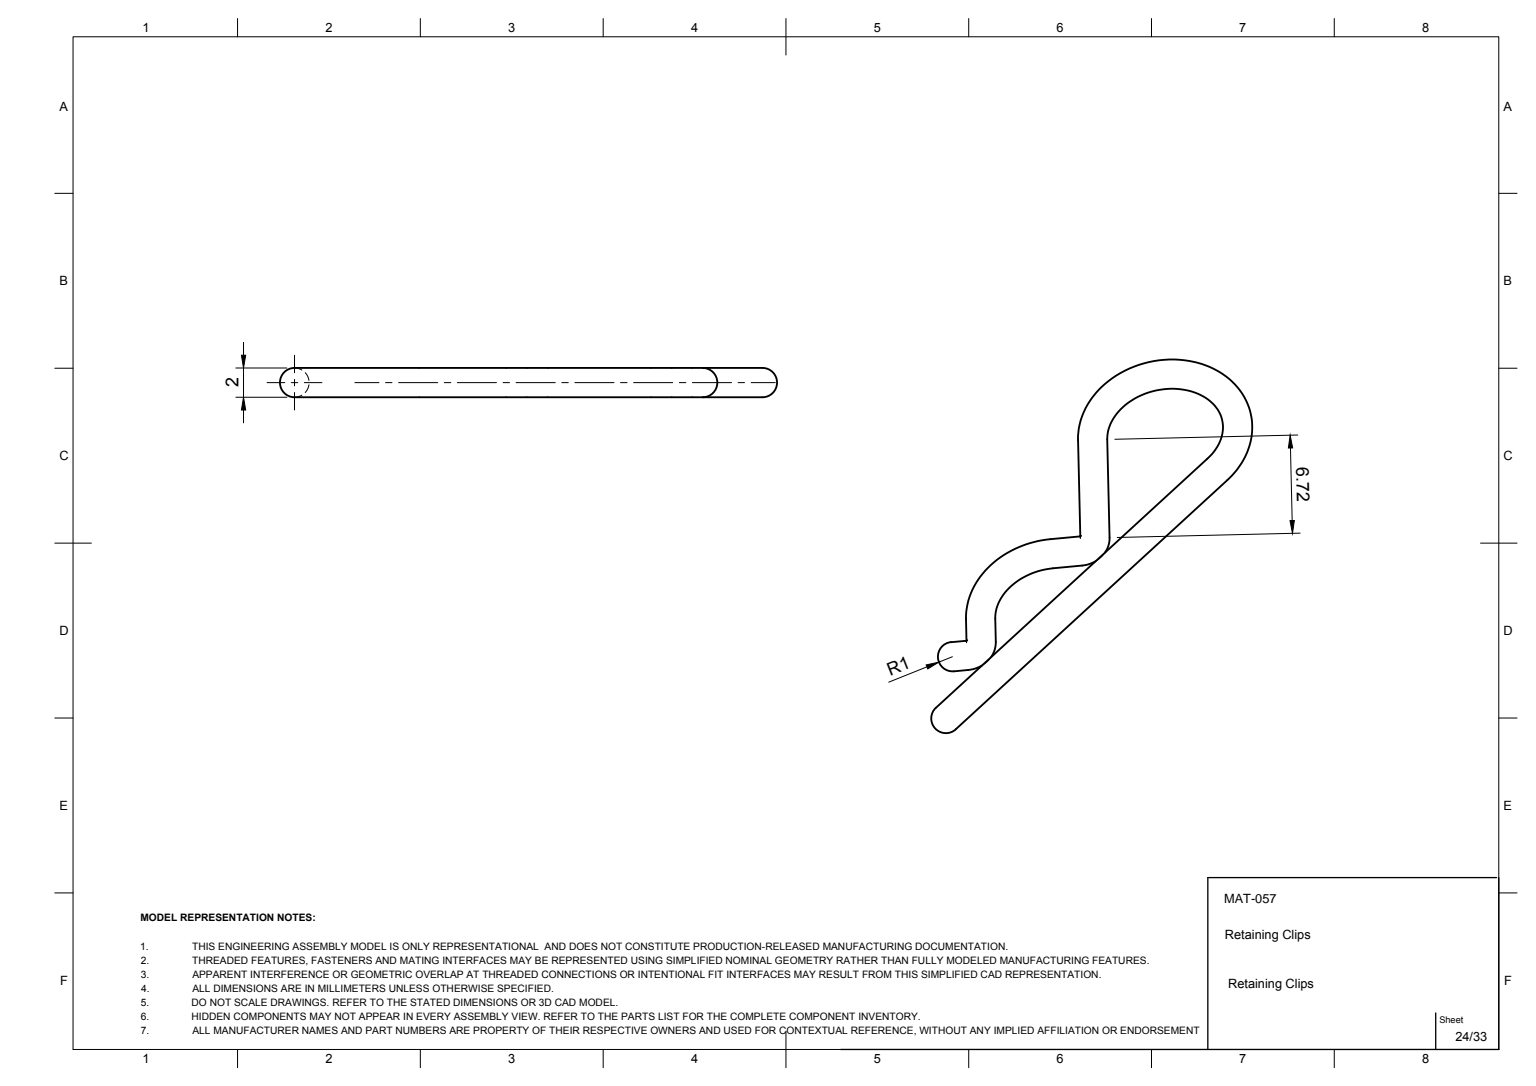
ISO-10303-21;
HEADER;
/* Generated by software containing ST-Developer
 * from STEP Tools, Inc. (www.steptools.com) 
 */

FILE_DESCRIPTION(
/* description */ ('STEP AP214', 'CAx-IF Rec.Pracs.---Representation and Presentation of Product Manufa
cturing Information (PMI)---4.0---2014-10-13'),
/* implementation_level */ '2;1');

FILE_NAME(
/* name */ 'Retaining Clips.step',
/* time_stamp */ '2026-10-28T23:34:22+01:00',
/* author */ (''),
/* organization */ (''),
/* preprocessor_version */ 'ST-DEVELOPER v20.2',
/* originating_system */ 'Autodesk Translation Framework v15.17.0.0',
/* authorisation */ '');

FILE_SCHEMA (('AP242_MANAGED_MODEL_BASED_3D_ENGINEERING_MIM_LF { 1 0 10303 442 2 1 4 }'));
ENDSEC;

DATA;
#10=MECHANICAL_DESIGN_GEOMETRIC_PRESENTATION_REPRESENTATION('',(#266,#267),#27807);
#219=SHAPE_REPRESENTATION_RELATIONSHIP('SRR','None',#27916,#241);
#241=ADVANCED_BREP_SHAPE_REPRESENTATION('',(#295,#296),#27796);
#266=STYLED_ITEM('',(#28070),#295);
#267=STYLED_ITEM('',(#28070),#296);
#295=MANIFOLD_SOLID_BREP('Body1',#12042);
#296=MANIFOLD_SOLID_BREP('Body2',#12043);
#318=(
BOUNDED_SURFACE()
B_SPLINE_SURFACE(2,2,((#22381,#22382,#22383),(#22384,#22385,#22386),(#22387,
#22388,#22389),(#22390,#22391,#22392),(#22393,#22394,#22395),(#22396,#22397,
#22398),(#22399,#22400,#22401),(#22402,#22403,#22404),(#22405,#22406,#22407)),
 .UNSPECIFIED.,.T.,.F.,.F.)
B_SPLINE_SURFACE_WITH_KNOTS((3,2,2,2,3),(3,3),(-3.14159265358979,-1.5707963267949,
0.,1.5707963267949,3.14159265358979),(-2.35619449019236,-0.785398163397175),
 .UNSPECIFIED.)
GEOMETRIC_REPRESENTATION_ITEM()
RATIONAL_B_SPLINE_SURFACE(((1.,0.707106781186444,1.),(0.707106781186499,
0.499999999999893,0.707106781186499),(1.,0.707106781186444,1.),(0.707106781186553,
0.499999999999931,0.707106781186553),(1.,0.707106781186444,1.),(0.707106781186499,
0.499999999999893,0.707106781186499),(1.,0.707106781186444,1.),(0.707106781186553,
0.499999999999931,0.707106781186553),(1.,0.707106781186444,1.)))
REPRESENTATION_ITEM('')
SURFACE()
);
#319=(
BOUNDED_SURFACE()
B_SPLINE_SURFACE(2,2,((#22408,#22409,#22410),(#22411,#22412,#22413),(#22414,
#22415,#22416),(#22417,#22418,#22419),(#22420,#22421,#22422),(#22423,#22424,
#22425),(#22426,#22427,#22428),(#22429,#22430,#22431),(#22432,#22433,#22434)),
 .UNSPECIFIED.,.T.,.F.,.F.)
B_SPLINE_SURFACE_WITH_KNOTS((3,2,2,2,3),(3,3),(-3.14159265358979,-1.5707963267949,
0.,1.5707963267949,3.14159265358979),(-2.35619449019277,-0.785398163397194),
 .UNSPECIFIED.)
GEOMETRIC_REPRESENTATION_ITEM()
RATIONAL_B_SPLINE_SURFACE(((1.,0.707106781186307,1.),(0.707106781186516,
0.499999999999808,0.707106781186516),(1.,0.707106781186307,1.),(0.707106781186497,
0.499999999999794,0.707106781186497),(1.,0.707106781186307,1.),(0.707106781186516,
0.499999999999808,0.707106781186516),(1.,0.707106781186307,1.),(0.707106781186497,
0.499999999999794,0.707106781186497),(1.,0.707106781186307,1.)))
REPRESENTATION_ITEM('')
SURFACE()
);
#320=(
BOUNDED_SURFACE()
B_SPLINE_SURFACE(2,2,((#22485,#22486,#22487),(#22488,#22489,#22490),(#22491,
#22492,#22493),(#22494,#22495,#22496),(#22497,#22498,#22499),(#22500,#22501,
#22502),(#22503,#22504,#22505),(#22506,#22507,#22508),(#22509,#22510,#22511)),
 .UNSPECIFIED.,.T.,.F.,.F.)
B_SPLINE_SURFACE_WITH_KNOTS((3,2,2,2,3),(3,3),(-3.14159265358979,-1.5707963267949,
0.,1.5707963267949,3.14159265358979),(-2.35619449019236,-0.785398163397439),
 .UNSPECIFIED.)
GEOMETRIC_REPRESENTATION_ITEM()
RATIONAL_B_SPLINE_SURFACE(((1.,0.707106781186539,1.),(0.707106781186531,
0.499999999999982,0.707106781186531),(1.,0.707106781186539,1.),(0.707106781186538,
0.499999999999987,0.707106781186538),(1.,0.707106781186539,1.),(0.707106781186531,
0.499999999999982,0.707106781186531),(1.,0.707106781186539,1.),(0.707106781186538,
0.499999999999987,0.707106781186538),(1.,0.707106781186539,1.)))
REPRESENTATION_ITEM('')
SURFACE()
);
#321=(
BOUNDED_SURFACE()
B_SPLINE_SURFACE(2,2,((#22512,#22513,#22514),(#22515,#22516,#22517),(#22518,
#22519,#22520),(#22521,#22522,#22523),(#22524,#22525,#22526),(#22527,#22528,
#22529),(#22530,#22531,#22532),(#22533,#22534,#22535),(#22536,#22537,#22538)),
 .UNSPECIFIED.,.T.,.F.,.F.)
B_SPLINE_SURFACE_WITH_KNOTS((3,2,2,2,3),(3,3),(-3.14159265358979,-1.5707963267949,
0.,1.5707963267949,3.14159265358979),(-2.35619449019241,-0.785398163397432),
 .UNSPECIFIED.)
GEOMETRIC_REPRESENTATION_ITEM()
RATIONAL_B_SPLINE_SURFACE(((1.,0.707106781186519,1.),(0.707106781186627,
0.500000000000036,0.707106781186627),(1.,0.707106781186519,1.),(0.707106781186571,
0.499999999999996,0.707106781186571),(1.,0.707106781186519,1.),(0.707106781186627,
0.500000000000036,0.707106781186627),(1.,0.707106781186519,1.),(0.707106781186571,
0.499999999999996,0.707106781186571),(1.,0.707106781186519,1.)))
REPRESENTATION_ITEM('')
SURFACE()
);
#331=SPHERICAL_SURFACE('',#13311,1.);
#332=SPHERICAL_SURFACE('',#13315,1.);
#333=SPHERICAL_SURFACE('',#13340,1.);
#334=SPHERICAL_SURFACE('',#13344,1.);
#834=TOROIDAL_SURFACE('',#13303,5.00000000000001,1.);
#835=TOROIDAL_SURFACE('',#13307,5.,1.);
#836=TOROIDAL_SURFACE('',#13332,5.00000000000001,1.);
#837=TOROIDAL_SURFACE('',#13336,5.,1.);
#1157=CYLINDRICAL_SURFACE('',#13319,0.999999999999997);
#1158=CYLINDRICAL_SURFACE('',#13322,0.999999999999983);
#1159=CYLINDRICAL_SURFACE('',#13325,0.999999999999997);
#1160=CYLINDRICAL_SURFACE('',#13328,1.00000000000002);
#1161=CYLINDRICAL_SURFACE('',#13331,1.00000000000002);
#1162=CYLINDRICAL_SURFACE('',#13348,1.);
#1163=CYLINDRICAL_SURFACE('',#13351,0.999999999999989);
#1164=CYLINDRICAL_SURFACE('',#13354,1.);
#1165=CYLINDRICAL_SURFACE('',#13357,0.999999999999999);
#1166=CYLINDRICAL_SURFACE('',#13360,0.999999999999993);
#1732=FACE_OUTER_BOUND('',#2510,.T.);
#1733=FACE_OUTER_BOUND('',#2511,.T.);
#1734=FACE_OUTER_BOUND('',#2512,.T.);
#1735=FACE_OUTER_BOUND('',#2513,.T.);
#1736=FACE_OUTER_BOUND('',#2514,.T.);
#1737=FACE_OUTER_BOUND('',#2515,.T.);
#1738=FACE_OUTER_BOUND('',#2516,.T.);
#1739=FACE_OUTER_BOUND('',#2517,.T.);
#1740=FACE_OUTER_BOUND('',#2518,.T.);
#1741=FACE_OUTER_BOUND('',#2519,.T.);
#1742=FACE_OUTER_BOUND('',#2520,.T.);
#1743=FACE_OUTER_BOUND('',#2521,.T.);
#1744=FACE_OUTER_BOUND('',#2522,.T.);
#1745=FACE_OUTER_BOUND('',#2523,.T.);
#1746=FACE_OUTER_BOUND('',#2524,.T.);
#1747=FACE_OUTER_BOUND('',#2525,.T.);
#1748=FACE_OUTER_BOUND('',#2526,.T.);
#1749=FACE_OUTER_BOUND('',#2527,.T.);
#1750=FACE_OUTER_BOUND('',#2528,.T.);
#1751=FACE_OUTER_BOUND('',#2529,.T.);
#1752=FACE_OUTER_BOUND('',#2530,.T.);
#1753=FACE_OUTER_BOUND('',#2531,.T.);
#2510=EDGE_LOOP('',(#10271,#10272,#10273,#10274));
#2511=EDGE_LOOP('',(#10275,#10276,#10277,#10278));
#2512=EDGE_LOOP('',(#10279,#10280,#10281,#10282));
#2513=EDGE_LOOP('',(#10283,#10284,#10285,#10286));
#2514=EDGE_LOOP('',(#10287,#10288,#10289,#10290,#10291,#10292));
#2515=EDGE_LOOP('',(#10293,#10294,#10295,#10296,#10297));
#2516=EDGE_LOOP('',(#10298,#10299,#10300,#10301,#10302));
#2517=EDGE_LOOP('',(#10303,#10304,#10305,#10306,#10307));
#2518=EDGE_LOOP('',(#10308,#10309,#10310,#10311,#10312));
#2519=EDGE_LOOP('',(#10313,#10314,#10315,#10316));
#2520=EDGE_LOOP('',(#10317,#10318,#10319,#10320));
#2521=EDGE_LOOP('',(#10321,#10322,#10323,#10324));
#2522=EDGE_LOOP('',(#10325,#10326,#10327,#10328));
#2523=EDGE_LOOP('',(#10329,#10330,#10331,#10332));
#2524=EDGE_LOOP('',(#10333,#10334,#10335,#10336));
#2525=EDGE_LOOP('',(#10337,#10338,#10339,#10340,#10341,#10342));
#2526=EDGE_LOOP('',(#10343,#10344,#10345,#10346,#10347));
#2527=EDGE_LOOP('',(#10348,#10349,#10350,#10351,#10352));
#2528=EDGE_LOOP('',(#10353,#10354,#10355,#10356,#10357));
#2529=EDGE_LOOP('',(#10358,#10359,#10360,#10361,#10362));
#2530=EDGE_LOOP('',(#10363,#10364,#10365,#10366));
#2531=EDGE_LOOP('',(#10367,#10368,#10369,#10370));
#3362=LINE('',#22359,#4182);
#3363=LINE('',#22366,#4183);
#3364=LINE('',#22370,#4184);
#3365=LINE('',#22377,#4185);
#3366=LINE('',#22380,#4186);
#3367=LINE('',#22463,#4187);
#3368=LINE('',#22470,#4188);
#3369=LINE('',#22474,#4189);
#3370=LINE('',#22481,#4190);
#3371=LINE('',#22484,#4191);
#4182=VECTOR('',#16384,0.999999999999997);
#4183=VECTOR('',#16393,0.999999999999983);
#4184=VECTOR('',#16398,0.999999999999997);
#4185=VECTOR('',#16407,1.00000000000002);
#4186=VECTOR('',#16412,1.00000000000002);
#4187=VECTOR('',#16447,1.);
#4188=VECTOR('',#16456,0.999999999999989);
#4189=VECTOR('',#16461,1.);
#4190=VECTOR('',#16470,0.999999999999999);
#4191=VECTOR('',#16475,0.999999999999993);
#4853=CIRCLE('',#13304,0.999999999999987);
#4854=CIRCLE('',#13305,4.00000000000001);
#4855=CIRCLE('',#13306,0.999999999999987);
#4856=CIRCLE('',#13308,0.999999999999987);
#4857=CIRCLE('',#13309,4.00000000000001);
#4858=CIRCLE('',#13310,0.999999999999987);
#4859=CIRCLE('',#13312,1.);
#4860=CIRCLE('',#13313,1.);
#4861=CIRCLE('',#13314,1.00000000000001);
#4862=CIRCLE('',#13316,1.00000000000002);
#4863=CIRCLE('',#13317,1.00000000000002);
#4864=CIRCLE('',#13318,0.999999999999996);
#4865=CIRCLE('',#13320,0.999999999999987);
#4866=CIRCLE('',#13321,0.999999999999987);
#4867=CIRCLE('',#13323,0.999999999999987);
#4868=CIRCLE('',#13324,0.999999999999987);
#4869=CIRCLE('',#13326,0.999999999999987);
#4870=CIRCLE('',#13327,0.999999999999987);
#4871=CIRCLE('',#13329,0.999999999999987);
#4872=CIRCLE('',#13330,0.999999999999987);
#4873=CIRCLE('',#13333,1.00000000000001);
#4874=CIRCLE('',#13334,4.);
#4875=CIRCLE('',#13335,1.00000000000001);
#4876=CIRCLE('',#13337,1.00000000000001);
#4877=CIRCLE('',#13338,4.);
#4878=CIRCLE('',#13339,1.00000000000001);
#4879=CIRCLE('',#13341,1.00000000000002);
#4880=CIRCLE('',#13342,1.00000000000002);
#4881=CIRCLE('',#13343,1.00000000000001);
#4882=CIRCLE('',#13345,0.999999999999993);
#4883=CIRCLE('',#13346,1.00000000000001);
#4884=CIRCLE('',#13347,0.999999999999993);
#4885=CIRCLE('',#13349,1.00000000000001);
#4886=CIRCLE('',#13350,1.00000000000001);
#4887=CIRCLE('',#13352,1.00000000000001);
#4888=CIRCLE('',#13353,1.00000000000001);
#4889=CIRCLE('',#13355,1.00000000000001);
#4890=CIRCLE('',#13356,1.00000000000001);
#4891=CIRCLE('',#13358,1.00000000000001);
#4892=CIRCLE('',#13359,1.00000000000001);
#5811=VERTEX_POINT('',#22332);
#5812=VERTEX_POINT('',#22334);
#5813=VERTEX_POINT('',#22338);
#5814=VERTEX_POINT('',#22340);
#5815=VERTEX_POINT('',#22344);
#5816=VERTEX_POINT('',#22345);
#5817=VERTEX_POINT('',#22348);
#5818=VERTEX_POINT('',#22351);
#5819=VERTEX_POINT('',#22352);
#5820=VERTEX_POINT('',#22355);
#5821=VERTEX_POINT('',#22358);
#5822=VERTEX_POINT('',#22360);
#5823=VERTEX_POINT('',#22364);
#5824=VERTEX_POINT('',#22369);
#5825=VERTEX_POINT('',#22371);
#5826=VERTEX_POINT('',#22375);
#5827=VERTEX_POINT('',#22436);
#5828=VERTEX_POINT('',#22438);
#5829=VERTEX_POINT('',#22442);
#5830=VERTEX_POINT('',#22444);
#5831=VERTEX_POINT('',#22448);
#5832=VERTEX_POINT('',#22449);
#5833=VERTEX_POINT('',#22452);
#5834=VERTEX_POINT('',#22455);
#5835=VERTEX_POINT('',#22456);
#5836=VERTEX_POINT('',#22458);
#5837=VERTEX_POINT('',#22462);
#5838=VERTEX_POINT('',#22464);
#5839=VERTEX_POINT('',#22468);
#5840=VERTEX_POINT('',#22473);
#5841=VERTEX_POINT('',#22475);
#5842=VERTEX_POINT('',#22479);
#7348=EDGE_CURVE('',#5811,#5811,#4853,.T.);
#7349=EDGE_CURVE('',#5811,#5812,#4854,.T.);
#7350=EDGE_CURVE('',#5812,#5812,#4855,.T.);
#7351=EDGE_CURVE('',#5813,#5813,#4856,.T.);
#7352=EDGE_CURVE('',#5813,#5814,#4857,.T.);
#7353=EDGE_CURVE('',#5814,#5814,#4858,.T.);
#7354=EDGE_CURVE('',#5815,#5816,#4859,.T.);
#7355=EDGE_CURVE('',#5816,#5815,#4860,.T.);
#7356=EDGE_CURVE('',#5816,#5817,#4861,.T.);
#7357=EDGE_CURVE('',#5818,#5819,#4862,.T.);
#7358=EDGE_CURVE('',#5819,#5818,#4863,.T.);
#7359=EDGE_CURVE('',#5820,#5819,#4864,.T.);
#7360=EDGE_CURVE('',#5815,#5821,#3362,.T.);
#7361=EDGE_CURVE('',#5822,#5821,#4865,.T.);
#7362=EDGE_CURVE('',#5821,#5822,#4866,.T.);
#7363=EDGE_CURVE('',#5822,#5823,#4867,.T.);
#7364=EDGE_CURVE('',#5823,#5811,#3363,.T.);
#7365=EDGE_CURVE('',#5823,#5822,#4868,.T.);
#7366=EDGE_CURVE('',#5812,#5824,#3364,.T.);
#7367=EDGE_CURVE('',#5825,#5824,#4869,.T.);
#7368=EDGE_CURVE('',#5824,#5825,#4870,.T.);
#7369=EDGE_CURVE('',#5825,#5826,#4871,.T.);
#7370=EDGE_CURVE('',#5826,#5813,#3365,.T.);
#7371=EDGE_CURVE('',#5826,#5825,#4872,.T.);
#7372=EDGE_CURVE('',#5814,#5818,#3366,.T.);
#7373=EDGE_CURVE('',#5827,#5827,#4873,.T.);
#7374=EDGE_CURVE('',#5827,#5828,#4874,.T.);
#7375=EDGE_CURVE('',#5828,#5828,#4875,.T.);
#7376=EDGE_CURVE('',#5829,#5829,#4876,.T.);
#7377=EDGE_CURVE('',#5829,#5830,#4877,.T.);
#7378=EDGE_CURVE('',#5830,#5830,#4878,.T.);
#7379=EDGE_CURVE('',#5831,#5832,#4879,.T.);
#7380=EDGE_CURVE('',#5832,#5831,#4880,.T.);
#7381=EDGE_CURVE('',#5833,#5832,#4881,.T.);
#7382=EDGE_CURVE('',#5834,#5835,#4882,.T.);
#7383=EDGE_CURVE('',#5836,#5834,#4883,.T.);
#7384=EDGE_CURVE('',#5835,#5834,#4884,.T.);
#7385=EDGE_CURVE('',#5831,#5837,#3367,.T.);
#7386=EDGE_CURVE('',#5838,#5837,#4885,.T.);
#7387=EDGE_CURVE('',#5837,#5838,#4886,.T.);
#7388=EDGE_CURVE('',#5838,#5839,#4887,.T.);
#7389=EDGE_CURVE('',#5839,#5827,#3368,.T.);
#7390=EDGE_CURVE('',#5839,#5838,#4888,.T.);
#7391=EDGE_CURVE('',#5828,#5840,#3369,.T.);
#7392=EDGE_CURVE('',#5841,#5840,#4889,.T.);
#7393=EDGE_CURVE('',#5840,#5841,#4890,.T.);
#7394=EDGE_CURVE('',#5841,#5842,#4891,.T.);
#7395=EDGE_CURVE('',#5842,#5829,#3370,.T.);
#7396=EDGE_CURVE('',#5842,#5841,#4892,.T.);
#7397=EDGE_CURVE('',#5830,#5835,#3371,.T.);
#10271=ORIENTED_EDGE('',*,*,#7348,.T.);
#10272=ORIENTED_EDGE('',*,*,#7349,.T.);
#10273=ORIENTED_EDGE('',*,*,#7350,.F.);
#10274=ORIENTED_EDGE('',*,*,#7349,.F.);
#10275=ORIENTED_EDGE('',*,*,#7351,.T.);
#10276=ORIENTED_EDGE('',*,*,#7352,.T.);
#10277=ORIENTED_EDGE('',*,*,#7353,.F.);
#10278=ORIENTED_EDGE('',*,*,#7352,.F.);
#10279=ORIENTED_EDGE('',*,*,#7354,.F.);
#10280=ORIENTED_EDGE('',*,*,#7355,.F.);
#10281=ORIENTED_EDGE('',*,*,#7356,.T.);
#10282=ORIENTED_EDGE('',*,*,#7356,.F.);
#10283=ORIENTED_EDGE('',*,*,#7357,.F.);
#10284=ORIENTED_EDGE('',*,*,#7358,.F.);
#10285=ORIENTED_EDGE('',*,*,#7359,.F.);
#10286=ORIENTED_EDGE('',*,*,#7359,.T.);
#10287=ORIENTED_EDGE('',*,*,#7354,.T.);
#10288=ORIENTED_EDGE('',*,*,#7355,.T.);
#10289=ORIENTED_EDGE('',*,*,#7360,.T.);
#10290=ORIENTED_EDGE('',*,*,#7361,.F.);
#10291=ORIENTED_EDGE('',*,*,#7362,.F.);
#10292=ORIENTED_EDGE('',*,*,#7360,.F.);
#10293=ORIENTED_EDGE('',*,*,#7363,.T.);
#10294=ORIENTED_EDGE('',*,*,#7364,.T.);
#10295=ORIENTED_EDGE('',*,*,#7348,.F.);
#10296=ORIENTED_EDGE('',*,*,#7364,.F.);
#10297=ORIENTED_EDGE('',*,*,#7365,.T.);
#10298=ORIENTED_EDGE('',*,*,#7350,.T.);
#10299=ORIENTED_EDGE('',*,*,#7366,.T.);
#10300=ORIENTED_EDGE('',*,*,#7367,.F.);
#10301=ORIENTED_EDGE('',*,*,#7368,.F.);
#10302=ORIENTED_EDGE('',*,*,#7366,.F.);
#10303=ORIENTED_EDGE('',*,*,#7369,.T.);
#10304=ORIENTED_EDGE('',*,*,#7370,.T.);
#10305=ORIENTED_EDGE('',*,*,#7351,.F.);
#10306=ORIENTED_EDGE('',*,*,#7370,.F.);
#10307=ORIENTED_EDGE('',*,*,#7371,.T.);
#10308=ORIENTED_EDGE('',*,*,#7353,.T.);
#10309=ORIENTED_EDGE('',*,*,#7372,.T.);
#10310=ORIENTED_EDGE('',*,*,#7357,.T.);
#10311=ORIENTED_EDGE('',*,*,#7358,.T.);
#10312=ORIENTED_EDGE('',*,*,#7372,.F.);
#10313=ORIENTED_EDGE('',*,*,#7361,.T.);
#10314=ORIENTED_EDGE('',*,*,#7362,.T.);
#10315=ORIENTED_EDGE('',*,*,#7365,.F.);
#10316=ORIENTED_EDGE('',*,*,#7363,.F.);
#10317=ORIENTED_EDGE('',*,*,#7367,.T.);
#10318=ORIENTED_EDGE('',*,*,#7368,.T.);
#10319=ORIENTED_EDGE('',*,*,#7371,.F.);
#10320=ORIENTED_EDGE('',*,*,#7369,.F.);
#10321=ORIENTED_EDGE('',*,*,#7373,.T.);
#10322=ORIENTED_EDGE('',*,*,#7374,.T.);
#10323=ORIENTED_EDGE('',*,*,#7375,.F.);
#10324=ORIENTED_EDGE('',*,*,#7374,.F.);
#10325=ORIENTED_EDGE('',*,*,#7376,.T.);
#10326=ORIENTED_EDGE('',*,*,#7377,.T.);
#10327=ORIENTED_EDGE('',*,*,#7378,.F.);
#10328=ORIENTED_EDGE('',*,*,#7377,.F.);
#10329=ORIENTED_EDGE('',*,*,#7379,.F.);
#10330=ORIENTED_EDGE('',*,*,#7380,.F.);
#10331=ORIENTED_EDGE('',*,*,#7381,.F.);
#10332=ORIENTED_EDGE('',*,*,#7381,.T.);
#10333=ORIENTED_EDGE('',*,*,#7382,.F.);
#10334=ORIENTED_EDGE('',*,*,#7383,.F.);
#10335=ORIENTED_EDGE('',*,*,#7383,.T.);
#10336=ORIENTED_EDGE('',*,*,#7384,.F.);
#10337=ORIENTED_EDGE('',*,*,#7379,.T.);
#10338=ORIENTED_EDGE('',*,*,#7380,.T.);
#10339=ORIENTED_EDGE('',*,*,#7385,.T.);
#10340=ORIENTED_EDGE('',*,*,#7386,.F.);
#10341=ORIENTED_EDGE('',*,*,#7387,.F.);
#10342=ORIENTED_EDGE('',*,*,#7385,.F.);
#10343=ORIENTED_EDGE('',*,*,#7388,.T.);
#10344=ORIENTED_EDGE('',*,*,#7389,.T.);
#10345=ORIENTED_EDGE('',*,*,#7373,.F.);
#10346=ORIENTED_EDGE('',*,*,#7389,.F.);
#10347=ORIENTED_EDGE('',*,*,#7390,.T.);
#10348=ORIENTED_EDGE('',*,*,#7375,.T.);
#10349=ORIENTED_EDGE('',*,*,#7391,.T.);
#10350=ORIENTED_EDGE('',*,*,#7392,.F.);
#10351=ORIENTED_EDGE('',*,*,#7393,.F.);
#10352=ORIENTED_EDGE('',*,*,#7391,.F.);
#10353=ORIENTED_EDGE('',*,*,#7394,.T.);
#10354=ORIENTED_EDGE('',*,*,#7395,.T.);
#10355=ORIENTED_EDGE('',*,*,#7376,.F.);
#10356=ORIENTED_EDGE('',*,*,#7395,.F.);
#10357=ORIENTED_EDGE('',*,*,#7396,.T.);
#10358=ORIENTED_EDGE('',*,*,#7378,.T.);
#10359=ORIENTED_EDGE('',*,*,#7397,.T.);
#10360=ORIENTED_EDGE('',*,*,#7384,.T.);
#10361=ORIENTED_EDGE('',*,*,#7382,.T.);
#10362=ORIENTED_EDGE('',*,*,#7397,.F.);
#10363=ORIENTED_EDGE('',*,*,#7386,.T.);
#10364=ORIENTED_EDGE('',*,*,#7387,.T.);
#10365=ORIENTED_EDGE('',*,*,#7390,.F.);
#10366=ORIENTED_EDGE('',*,*,#7388,.F.);
#10367=ORIENTED_EDGE('',*,*,#7392,.T.);
#10368=ORIENTED_EDGE('',*,*,#7393,.T.);
#10369=ORIENTED_EDGE('',*,*,#7396,.F.);
#10370=ORIENTED_EDGE('',*,*,#7394,.F.);
#11814=ADVANCED_FACE('',(#1732),#834,.T.);
#11815=ADVANCED_FACE('',(#1733),#835,.T.);
#11816=ADVANCED_FACE('',(#1734),#331,.T.);
#11817=ADVANCED_FACE('',(#1735),#332,.T.);
#11818=ADVANCED_FACE('',(#1736),#1157,.T.);
#11819=ADVANCED_FACE('',(#1737),#1158,.T.);
#11820=ADVANCED_FACE('',(#1738),#1159,.T.);
#11821=ADVANCED_FACE('',(#1739),#1160,.T.);
#11822=ADVANCED_FACE('',(#1740),#1161,.T.);
#11823=ADVANCED_FACE('',(#1741),#318,.F.);
#11824=ADVANCED_FACE('',(#1742),#319,.F.);
#11825=ADVANCED_FACE('',(#1743),#836,.T.);
#11826=ADVANCED_FACE('',(#1744),#837,.T.);
#11827=ADVANCED_FACE('',(#1745),#333,.T.);
#11828=ADVANCED_FACE('',(#1746),#334,.T.);
#11829=ADVANCED_FACE('',(#1747),#1162,.T.);
#11830=ADVANCED_FACE('',(#1748),#1163,.T.);
#11831=ADVANCED_FACE('',(#1749),#1164,.T.);
#11832=ADVANCED_FACE('',(#1750),#1165,.T.);
#11833=ADVANCED_FACE('',(#1751),#1166,.T.);
#11834=ADVANCED_FACE('',(#1752),#320,.F.);
#11835=ADVANCED_FACE('',(#1753),#321,.F.);
#12042=CLOSED_SHELL('',(#11814,#11815,#11816,#11817,#11818,#11819,#11820,
#11821,#11822,#11823,#11824));
#12043=CLOSED_SHELL('',(#11825,#11826,#11827,#11828,#11829,#11830,#11831,
#11832,#11833,#11834,#11835));
#13302=AXIS2_PLACEMENT_3D('',#22330,#16348,#16349);
#13303=AXIS2_PLACEMENT_3D('',#22331,#16350,#16351);
#13304=AXIS2_PLACEMENT_3D('',#22333,#16352,#16353);
#13305=AXIS2_PLACEMENT_3D('',#22335,#16354,#16355);
#13306=AXIS2_PLACEMENT_3D('',#22336,#16356,#16357);
#13307=AXIS2_PLACEMENT_3D('',#22337,#16358,#16359);
#13308=AXIS2_PLACEMENT_3D('',#22339,#16360,#16361);
#13309=AXIS2_PLACEMENT_3D('',#22341,#16362,#16363);
#13310=AXIS2_PLACEMENT_3D('',#22342,#16364,#16365);
#13311=AXIS2_PLACEMENT_3D('',#22343,#16366,#16367);
#13312=AXIS2_PLACEMENT_3D('',#22346,#16368,#16369);
#13313=AXIS2_PLACEMENT_3D('',#22347,#16370,#16371);
#13314=AXIS2_PLACEMENT_3D('',#22349,#16372,#16373);
#13315=AXIS2_PLACEMENT_3D('',#22350,#16374,#16375);
#13316=AXIS2_PLACEMENT_3D('',#22353,#16376,#16377);
#13317=AXIS2_PLACEMENT_3D('',#22354,#16378,#16379);
#13318=AXIS2_PLACEMENT_3D('',#22356,#16380,#16381);
#13319=AXIS2_PLACEMENT_3D('',#22357,#16382,#16383);
#13320=AXIS2_PLACEMENT_3D('',#22361,#16385,#16386);
#13321=AXIS2_PLACEMENT_3D('',#22362,#16387,#16388);
#13322=AXIS2_PLACEMENT_3D('',#22363,#16389,#16390);
#13323=AXIS2_PLACEMENT_3D('',#22365,#16391,#16392);
#13324=AXIS2_PLACEMENT_3D('',#22367,#16394,#16395);
#13325=AXIS2_PLACEMENT_3D('',#22368,#16396,#16397);
#13326=AXIS2_PLACEMENT_3D('',#22372,#16399,#16400);
#13327=AXIS2_PLACEMENT_3D('',#22373,#16401,#16402);
#13328=AXIS2_PLACEMENT_3D('',#22374,#16403,#16404);
#13329=AXIS2_PLACEMENT_3D('',#22376,#16405,#16406);
#13330=AXIS2_PLACEMENT_3D('',#22378,#16408,#16409);
#13331=AXIS2_PLACEMENT_3D('',#22379,#16410,#16411);
#13332=AXIS2_PLACEMENT_3D('',#22435,#16413,#16414);
#13333=AXIS2_PLACEMENT_3D('',#22437,#16415,#16416);
#13334=AXIS2_PLACEMENT_3D('',#22439,#16417,#16418);
#13335=AXIS2_PLACEMENT_3D('',#22440,#16419,#16420);
#13336=AXIS2_PLACEMENT_3D('',#22441,#16421,#16422);
#13337=AXIS2_PLACEMENT_3D('',#22443,#16423,#16424);
#13338=AXIS2_PLACEMENT_3D('',#22445,#16425,#16426);
#13339=AXIS2_PLACEMENT_3D('',#22446,#16427,#16428);
#13340=AXIS2_PLACEMENT_3D('',#22447,#16429,#16430);
#13341=AXIS2_PLACEMENT_3D('',#22450,#16431,#16432);
#13342=AXIS2_PLACEMENT_3D('',#22451,#16433,#16434);
#13343=AXIS2_PLACEMENT_3D('',#22453,#16435,#16436);
#13344=AXIS2_PLACEMENT_3D('',#22454,#16437,#16438);
#13345=AXIS2_PLACEMENT_3D('',#22457,#16439,#16440);
#13346=AXIS2_PLACEMENT_3D('',#22459,#16441,#16442);
#13347=AXIS2_PLACEMENT_3D('',#22460,#16443,#16444);
#13348=AXIS2_PLACEMENT_3D('',#22461,#16445,#16446);
#13349=AXIS2_PLACEMENT_3D('',#22465,#16448,#16449);
#13350=AXIS2_PLACEMENT_3D('',#22466,#16450,#16451);
#13351=AXIS2_PLACEMENT_3D('',#22467,#16452,#16453);
#13352=AXIS2_PLACEMENT_3D('',#22469,#16454,#16455);
#13353=AXIS2_PLACEMENT_3D('',#22471,#16457,#16458);
#13354=AXIS2_PLACEMENT_3D('',#22472,#16459,#16460);
#13355=AXIS2_PLACEMENT_3D('',#22476,#16462,#16463);
#13356=AXIS2_PLACEMENT_3D('',#22477,#16464,#16465);
#13357=AXIS2_PLACEMENT_3D('',#22478,#16466,#16467);
#13358=AXIS2_PLACEMENT_3D('',#22480,#16468,#16469);
#13359=AXIS2_PLACEMENT_3D('',#22482,#16471,#16472);
#13360=AXIS2_PLACEMENT_3D('',#22483,#16473,#16474);
#16348=DIRECTION('axis',(0.,0.,1.));
#16349=DIRECTION('refdir',(1.,0.,0.));
#16350=DIRECTION('center_axis',(-0.179306265355413,-0.00912071322752245,
0.983751023274952));
#16351=DIRECTION('ref_axis',(-0.0508009940819341,0.998708795896125,0.));
#16352=DIRECTION('center_axis',(-0.7306405634129,0.670855725914997,-0.126952597857399));
#16353=DIRECTION('ref_axis',(-0.179306265355412,-0.00912071322752053,0.983751023274952));
#16354=DIRECTION('center_axis',(0.179306265355413,0.00912071322752245,-0.983751023274952));
#16355=DIRECTION('ref_axis',(-0.0508009940819232,0.998708795896125,7.43409742643818E-16));
#16356=DIRECTION('center_axis',(0.658797108600206,0.741531798102594,0.1269525978574));
#16357=DIRECTION('ref_axis',(-0.179306265355399,-0.00912071322753601,0.983751023274955));
#16358=DIRECTION('center_axis',(-0.179306265355413,-0.00912071322752245,
0.983751023274952));
#16359=DIRECTION('ref_axis',(-0.0508009940819344,0.998708795896125,0.));
#16360=DIRECTION('center_axis',(-0.730640563412892,0.670855725915006,-0.126952597857398));
#16361=DIRECTION('ref_axis',(-0.179306265355412,-0.00912071322752053,0.983751023274952));
#16362=DIRECTION('center_axis',(0.179306265355413,0.00912071322752245,-0.983751023274952));
#16363=DIRECTION('ref_axis',(-0.0508009940819232,0.998708795896125,7.43409742643818E-16));
#16364=DIRECTION('center_axis',(0.0508009940819268,-0.998708795896125,-7.81461095279302E-17));
#16365=DIRECTION('ref_axis',(-0.179306265355397,-0.00912071322752166,0.983751023274955));
#16366=DIRECTION('center_axis',(0.,0.,1.));
#16367=DIRECTION('ref_axis',(1.,0.,0.));
#16368=DIRECTION('center_axis',(0.658797108600203,0.741531798102596,0.126952597857399));
#16369=DIRECTION('ref_axis',(-0.730640563412887,0.670855725915008,-0.126952597857418));
#16370=DIRECTION('center_axis',(0.658797108600203,0.741531798102596,0.126952597857399));
#16371=DIRECTION('ref_axis',(-0.730640563412887,0.670855725915008,-0.126952597857418));
#16372=DIRECTION('center_axis',(0.,-1.,0.));
#16373=DIRECTION('ref_axis',(-1.,0.,0.));
#16374=DIRECTION('center_axis',(1.,0.,0.));
#16375=DIRECTION('ref_axis',(0.,-1.,0.));
#16376=DIRECTION('center_axis',(-0.0508009940819267,0.998708795896125,1.00133183721819E-16));
#16377=DIRECTION('ref_axis',(0.98248079991651,0.0499755299114802,0.17953808566842));
#16378=DIRECTION('center_axis',(-0.0508009940819267,0.998708795896125,1.00133183721819E-16));
#16379=DIRECTION('ref_axis',(0.98248079991651,0.0499755299114802,0.17953808566842));
#16380=DIRECTION('center_axis',(0.,0.,1.));
#16381=DIRECTION('ref_axis',(0.,1.,0.));
#16382=DIRECTION('center_axis',(-0.658797108600203,-0.741531798102596,-0.126952597857399));
#16383=DIRECTION('ref_axis',(-0.730640563412892,0.670855725915008,-0.126952597857391));
#16384=DIRECTION('',(0.658797108600203,0.741531798102596,0.126952597857399));
#16385=DIRECTION('center_axis',(0.658797108600207,0.741531798102593,0.1269525978574));
#16386=DIRECTION('ref_axis',(-0.179306265355399,-0.00912071322753602,0.983751023274955));
#16387=DIRECTION('center_axis',(0.658797108600207,0.741531798102593,0.1269525978574));
#16388=DIRECTION('ref_axis',(-0.179306265355399,-0.00912071322753602,0.983751023274955));
#16389=DIRECTION('center_axis',(0.730640563412901,-0.670855725914996,0.126952597857399));
#16390=DIRECTION('ref_axis',(-0.658797108600193,-0.741531798102606,-0.126952597857392));
#16391=DIRECTION('center_axis',(-0.730640563412901,0.670855725914996,-0.126952597857399));
#16392=DIRECTION('ref_axis',(-0.179306265355412,-0.00912071322752052,0.983751023274952));
#16393=DIRECTION('',(-0.730640563412901,0.670855725914996,-0.126952597857399));
#16394=DIRECTION('center_axis',(-0.730640563412901,0.670855725914996,-0.126952597857399));
#16395=DIRECTION('ref_axis',(-0.179306265355412,-0.00912071322752052,0.983751023274952));
#16396=DIRECTION('center_axis',(-0.658797108600206,-0.741531798102594,-0.1269525978574));
#16397=DIRECTION('ref_axis',(-0.73064056341289,0.67085572591501,-0.126952597857391));
#16398=DIRECTION('',(0.658797108600206,0.741531798102594,0.1269525978574));
#16399=DIRECTION('center_axis',(0.658797108600204,0.741531798102595,0.126952597857399));
#16400=DIRECTION('ref_axis',(-0.179306265355399,-0.00912071322753602,0.983751023274955));
#16401=DIRECTION('center_axis',(0.658797108600204,0.741531798102595,0.126952597857399));
#16402=DIRECTION('ref_axis',(-0.179306265355399,-0.00912071322753602,0.983751023274955));
#16403=DIRECTION('center_axis',(0.730640563412891,-0.670855725915007,0.126952597857398));
#16404=DIRECTION('ref_axis',(-0.658797108600205,-0.741531798102597,-0.126952597857384));
#16405=DIRECTION('center_axis',(-0.730640563412891,0.670855725915007,-0.126952597857398));
#16406=DIRECTION('ref_axis',(-0.179306265355412,-0.00912071322752052,0.983751023274952));
#16407=DIRECTION('',(-0.730640563412891,0.670855725915007,-0.126952597857398));
#16408=DIRECTION('center_axis',(-0.730640563412891,0.670855725915007,-0.126952597857398));
#16409=DIRECTION('ref_axis',(-0.179306265355412,-0.00912071322752052,0.983751023274952));
#16410=DIRECTION('center_axis',(-0.0508009940819267,0.998708795896125,1.00133183721819E-16));
#16411=DIRECTION('ref_axis',(0.98248079991651,0.0499755299114802,0.17953808566842));
#16412=DIRECTION('',(0.0508009940819267,-0.998708795896125,-1.00133183721819E-16));
#16413=DIRECTION('center_axis',(-0.628842175749928,0.599591913317124,0.49502227776415));
#16414=DIRECTION('ref_axis',(-0.690074255005139,-0.723738573366864,0.));
#16415=DIRECTION('center_axis',(-0.234623360105886,-0.753309635298807,0.614391139469477));
#16416=DIRECTION('ref_axis',(-0.628842175749927,0.599591913317124,0.495022277764151));
#16417=DIRECTION('center_axis',(0.628842175749928,-0.599591913317124,-0.49502227776415));
#16418=DIRECTION('ref_axis',(-0.69007425500514,-0.723738573366862,5.49585130476149E-16));
#16419=DIRECTION('center_axis',(-0.741289010366885,-0.270211270769156,-0.614391139469478));
#16420=DIRECTION('ref_axis',(-0.628842175749928,0.599591913317122,0.495022277764152));
#16421=DIRECTION('center_axis',(-0.628842175749928,0.599591913317124,0.49502227776415));
#16422=DIRECTION('ref_axis',(-0.690074255005139,-0.723738573366864,0.));
#16423=DIRECTION('center_axis',(-0.234623360105896,-0.75330963529881,0.614391139469469));
#16424=DIRECTION('ref_axis',(-0.628842175749927,0.599591913317124,0.495022277764151));
#16425=DIRECTION('center_axis',(0.628842175749928,-0.599591913317124,-0.49502227776415));
#16426=DIRECTION('ref_axis',(-0.69007425500514,-0.723738573366862,5.49585130476149E-16));
#16427=DIRECTION('center_axis',(0.69007425500514,0.723738573366862,-1.81566217392232E-16));
#16428=DIRECTION('ref_axis',(-0.628842175749927,0.599591913317123,0.495022277764153));
#16429=DIRECTION('center_axis',(0.,0.,1.));
#16430=DIRECTION('ref_axis',(1.,0.,0.));
#16431=DIRECTION('center_axis',(-0.741289010366885,-0.270211270769158,-0.614391139469476));
#16432=DIRECTION('ref_axis',(-0.234623360105902,-0.753309635298806,0.614391139469472));
#16433=DIRECTION('center_axis',(-0.741289010366885,-0.270211270769158,-0.614391139469476));
#16434=DIRECTION('ref_axis',(-0.234623360105902,-0.753309635298806,0.614391139469472));
#16435=DIRECTION('center_axis',(0.,-1.,0.));
#16436=DIRECTION('ref_axis',(-1.,0.,0.));
#16437=DIRECTION('center_axis',(1.,0.,0.));
#16438=DIRECTION('ref_axis',(0.,-1.,0.));
#16439=DIRECTION('center_axis',(-0.69007425500514,-0.723738573366862,7.51590717680294E-17));
#16440=DIRECTION('ref_axis',(-0.358266717093849,0.341602129539051,-0.868880282039581));
#16441=DIRECTION('center_axis',(0.,0.,1.));
#16442=DIRECTION('ref_axis',(0.,1.,0.));
#16443=DIRECTION('center_axis',(-0.69007425500514,-0.723738573366862,7.51590717680294E-17));
#16444=DIRECTION('ref_axis',(-0.358266717093849,0.341602129539051,-0.868880282039581));
#16445=DIRECTION('center_axis',(0.741289010366885,0.270211270769158,0.614391139469476));
#16446=DIRECTION('ref_axis',(-0.234623360105893,-0.753309635298815,0.614391139469465));
#16447=DIRECTION('',(-0.741289010366885,-0.270211270769158,-0.614391139469476));
#16448=DIRECTION('center_axis',(-0.741289010366884,-0.270211270769154,-0.614391139469479));
#16449=DIRECTION('ref_axis',(-0.628842175749928,0.599591913317122,0.495022277764152));
#16450=DIRECTION('center_axis',(-0.741289010366884,-0.270211270769154,-0.614391139469479));
#16451=DIRECTION('ref_axis',(-0.628842175749928,0.599591913317122,0.495022277764152));
#16452=DIRECTION('center_axis',(0.234623360105886,0.753309635298807,-0.614391139469477));
#16453=DIRECTION('ref_axis',(0.741289010366886,0.270211270769172,0.614391139469469));
#16454=DIRECTION('center_axis',(-0.234623360105886,-0.753309635298807,0.614391139469477));
#16455=DIRECTION('ref_axis',(-0.628842175749927,0.599591913317124,0.495022277764151));
#16456=DIRECTION('',(-0.234623360105886,-0.753309635298807,0.614391139469477));
#16457=DIRECTION('center_axis',(-0.234623360105886,-0.753309635298807,0.614391139469477));
#16458=DIRECTION('ref_axis',(-0.628842175749927,0.599591913317124,0.495022277764151));
#16459=DIRECTION('center_axis',(0.741289010366884,0.270211270769155,0.614391139469478));
#16460=DIRECTION('ref_axis',(-0.234623360105895,-0.753309635298815,0.614391139469463));
#16461=DIRECTION('',(-0.741289010366885,-0.270211270769155,-0.614391139469478));
#16462=DIRECTION('center_axis',(-0.741289010366885,-0.270211270769157,-0.614391139469477));
#16463=DIRECTION('ref_axis',(-0.628842175749928,0.599591913317122,0.495022277764152));
#16464=DIRECTION('center_axis',(-0.741289010366885,-0.270211270769157,-0.614391139469477));
#16465=DIRECTION('ref_axis',(-0.628842175749928,0.599591913317122,0.495022277764152));
#16466=DIRECTION('center_axis',(0.234623360105896,0.75330963529881,-0.614391139469469));
#16467=DIRECTION('ref_axis',(0.741289010366884,0.27021127076916,0.614391139469476));
#16468=DIRECTION('center_axis',(-0.234623360105896,-0.75330963529881,0.614391139469469));
#16469=DIRECTION('ref_axis',(-0.628842175749927,0.599591913317124,0.495022277764151));
#16470=DIRECTION('',(-0.234623360105896,-0.75330963529881,0.614391139469469));
#16471=DIRECTION('center_axis',(-0.234623360105896,-0.75330963529881,0.614391139469469));
#16472=DIRECTION('ref_axis',(-0.628842175749927,0.599591913317124,0.495022277764151));
#16473=DIRECTION('center_axis',(-0.69007425500514,-0.723738573366862,7.51590717680294E-17));
#16474=DIRECTION('ref_axis',(-0.358266717093849,0.341602129539051,-0.868880282039581));
#16475=DIRECTION('',(0.69007425500514,0.723738573366862,-7.51590717680294E-17));
#22330=CARTESIAN_POINT('',(0.,0.,0.));
#22331=CARTESIAN_POINT('Origin',(272.351065622502,161.693151647739,245.488927842219));
#22332=CARTESIAN_POINT('',(269.715877188101,158.727024455329,244.98111745079));
#22333=CARTESIAN_POINT('Origin',(269.057080079501,157.985492657226,244.854164852932));
#22334=CARTESIAN_POINT('',(269.42850336885,164.376574551399,244.98111745079));
#22335=CARTESIAN_POINT('Origin',(272.351065622502,161.693151647739,245.488927842219));
#22336=CARTESIAN_POINT('Origin',(268.697862805437,165.047430277314,244.854164852932));
#22337=CARTESIAN_POINT('Origin',(267.097176680551,177.288521295714,244.675902705153));
#22338=CARTESIAN_POINT('',(264.46198824615,174.322394103304,244.168092313724));
#22339=CARTESIAN_POINT('Origin',(263.80319113755,173.580862305201,244.041139715866));
#22340=CARTESIAN_POINT('',(271.027099880217,177.48842341536,245.394055047827));
#22341=CARTESIAN_POINT('Origin',(267.097176680551,177.288521295714,244.675902705153));
#22342=CARTESIAN_POINT('Origin',(272.009580680134,177.538398945271,245.573593133495));
#22343=CARTESIAN_POINT('Origin',(269.931407552539,154.489861883276,244.98111745079));
#22344=CARTESIAN_POINT('',(270.662048115952,153.819006157361,245.108070048647));
#22345=CARTESIAN_POINT('',(269.742185248056,154.489861883276,245.963051725314));
#22346=CARTESIAN_POINT('Origin',(269.931407552539,154.489861883276,244.98111745079));
#22347=CARTESIAN_POINT('Origin',(269.931407552539,154.489861883276,244.98111745079));
#22348=CARTESIAN_POINT('',(269.931407552539,154.489861883276,243.98111745079));
#22349=CARTESIAN_POINT('Origin',(269.931407552539,154.489861883276,244.98111745079));
#22350=CARTESIAN_POINT('Origin',(273.381207520346,150.573261456076,245.573593133495));
#22351=CARTESIAN_POINT('',(272.398726720429,150.523285926165,245.394055047827));
#22352=CARTESIAN_POINT('',(274.379916316242,150.624062450158,245.573593133495));
#22353=CARTESIAN_POINT('Origin',(273.381207520346,150.573261456076,245.573593133495));
#22354=CARTESIAN_POINT('Origin',(273.381207520346,150.573261456076,245.573593133495));
#22355=CARTESIAN_POINT('',(274.381207520346,150.573261456076,245.573593133495));
#22356=CARTESIAN_POINT('Origin',(273.381207520346,150.573261456076,245.573593133495));
#22357=CARTESIAN_POINT('Origin',(270.590204661139,155.231393681379,245.108070048647));
#22358=CARTESIAN_POINT('',(271.320845224552,154.560537955464,245.235022646504));
#22359=CARTESIAN_POINT('',(271.320845224552,154.560537955464,245.235022646504));
#22360=CARTESIAN_POINT('',(269.859564097726,155.902249407294,244.98111745079));
#22361=CARTESIAN_POINT('Origin',(270.590204661139,155.231393681379,245.108070048647));
#22362=CARTESIAN_POINT('Origin',(270.590204661139,155.231393681379,245.108070048647));
#22363=CARTESIAN_POINT('Origin',(269.057080079501,157.985492657226,244.854164852932));
#22364=CARTESIAN_POINT('',(271.177158314927,157.385313003499,245.235022646504));
#22365=CARTESIAN_POINT('Origin',(270.518361206326,156.643781205396,245.108070048647));
#22366=CARTESIAN_POINT('',(269.715877188101,158.727024455329,244.98111745079));
#22367=CARTESIAN_POINT('Origin',(270.518361206326,156.643781205396,245.108070048647));
#22368=CARTESIAN_POINT('Origin',(270.015457022638,166.530493873519,245.108070048647));
#22369=CARTESIAN_POINT('',(270.74609758605,165.859638147604,245.235022646504));
#22370=CARTESIAN_POINT('',(270.74609758605,165.859638147604,245.235022646504));
#22371=CARTESIAN_POINT('',(269.284816459225,167.201349599434,244.98111745079));
#22372=CARTESIAN_POINT('Origin',(270.015457022638,166.530493873519,245.108070048647));
#22373=CARTESIAN_POINT('Origin',(270.015457022638,166.530493873519,245.108070048647));
#22374=CARTESIAN_POINT('Origin',(263.80319113755,173.580862305201,244.041139715866));
#22375=CARTESIAN_POINT('',(270.602410676425,168.68441319564,245.235022646504));
#22376=CARTESIAN_POINT('Origin',(269.943613567825,167.942881397537,245.108070048647));
#22377=CARTESIAN_POINT('',(264.46198824615,174.322394103304,244.168092313724));
#22378=CARTESIAN_POINT('Origin',(269.943613567825,167.942881397537,245.108070048647));
#22379=CARTESIAN_POINT('Origin',(273.432008514428,149.57455266018,245.573593133495));
#22380=CARTESIAN_POINT('',(272.449527714511,149.524577130268,245.394055047827));
#22381=CARTESIAN_POINT('Ctrl Pts',(269.859564097726,155.902249407293,244.98111745079));
#22382=CARTESIAN_POINT('Ctrl Pts',(269.859564097726,155.902249407293,244.98111745079));
#22383=CARTESIAN_POINT('Ctrl Pts',(269.859564097726,155.902249407294,244.98111745079));
#22384=CARTESIAN_POINT('Ctrl Pts',(269.680257832371,155.893128694066,245.964868474065));
#22385=CARTESIAN_POINT('Ctrl Pts',(269.680257832371,155.893128694066,245.964868474065));
#22386=CARTESIAN_POINT('Ctrl Pts',(269.680257832371,155.893128694066,245.964868474065));
#22387=CARTESIAN_POINT('Ctrl Pts',(270.339054940971,156.634660492169,246.091821071922));
#22388=CARTESIAN_POINT('Ctrl Pts',(271.069695504384,155.963804766254,246.218773669779));
#22389=CARTESIAN_POINT('Ctrl Pts',(270.410898395784,155.222272968151,246.091821071922));
#22390=CARTESIAN_POINT('Ctrl Pts',(270.997852049571,157.376192290271,246.218773669779));
#22391=CARTESIAN_POINT('Ctrl Pts',(272.459133176397,156.034480838441,246.472678865494));
#22392=CARTESIAN_POINT('Ctrl Pts',(271.141538959196,154.551417242236,246.218773669779));
#22393=CARTESIAN_POINT('Ctrl Pts',(271.177158314927,157.385313003499,245.235022646504));
#22394=CARTESIAN_POINT('Ctrl Pts',(272.638439441753,156.043601551669,245.488927842219));
#22395=CARTESIAN_POINT('Ctrl Pts',(271.320845224552,154.560537955463,245.235022646504));
#22396=CARTESIAN_POINT('Ctrl Pts',(271.356464580282,157.394433716726,244.251271623229));
#22397=CARTESIAN_POINT('Ctrl Pts',(272.817745707108,156.052722264896,244.505176818944));
#22398=CARTESIAN_POINT('Ctrl Pts',(271.500151489907,154.569658668691,244.251271623229));
#22399=CARTESIAN_POINT('Ctrl Pts',(270.697667471682,156.652901918624,244.124319025372));
#22400=CARTESIAN_POINT('Ctrl Pts',(271.428308035095,155.982046192709,244.251271623229));
#22401=CARTESIAN_POINT('Ctrl Pts',(270.769510926494,155.240514394606,244.124319025372));
#22402=CARTESIAN_POINT('Ctrl Pts',(270.038870363082,155.911370120521,243.997366427515));
#22403=CARTESIAN_POINT('Ctrl Pts',(270.038870363082,155.911370120521,243.997366427515));
#22404=CARTESIAN_POINT('Ctrl Pts',(270.038870363082,155.911370120521,243.997366427515));
#22405=CARTESIAN_POINT('Ctrl Pts',(269.859564097726,155.902249407293,244.98111745079));
#22406=CARTESIAN_POINT('Ctrl Pts',(269.859564097726,155.902249407293,244.98111745079));
#22407=CARTESIAN_POINT('Ctrl Pts',(269.859564097726,155.902249407294,244.98111745079));
#22408=CARTESIAN_POINT('Ctrl Pts',(269.284816459225,167.201349599434,244.98111745079));
#22409=CARTESIAN_POINT('Ctrl Pts',(269.284816459225,167.201349599434,244.98111745079));
#22410=CARTESIAN_POINT('Ctrl Pts',(269.284816459225,167.201349599434,244.98111745079));
#22411=CARTESIAN_POINT('Ctrl Pts',(269.105510193869,167.192228886207,245.964868474065));
#22412=CARTESIAN_POINT('Ctrl Pts',(269.105510193869,167.192228886207,245.964868474065));
#22413=CARTESIAN_POINT('Ctrl Pts',(269.105510193869,167.192228886207,245.964868474065));
#22414=CARTESIAN_POINT('Ctrl Pts',(269.764307302469,167.93376068431,246.091821071922));
#22415=CARTESIAN_POINT('Ctrl Pts',(270.494947865883,167.262904958394,246.218773669779));
#22416=CARTESIAN_POINT('Ctrl Pts',(269.836150757282,166.521373160292,246.091821071922));
#22417=CARTESIAN_POINT('Ctrl Pts',(270.423104411069,168.675292482413,246.218773669779));
#22418=CARTESIAN_POINT('Ctrl Pts',(271.884385537896,167.333581030582,246.472678865494));
#22419=CARTESIAN_POINT('Ctrl Pts',(270.566791320695,165.850517434376,246.218773669779));
#22420=CARTESIAN_POINT('Ctrl Pts',(270.602410676424,168.68441319564,245.235022646504));
#22421=CARTESIAN_POINT('Ctrl Pts',(272.063691803252,167.34270174381,245.488927842219));
#22422=CARTESIAN_POINT('Ctrl Pts',(270.74609758605,165.859638147604,245.235022646504));
#22423=CARTESIAN_POINT('Ctrl Pts',(270.78171694178,168.693533908868,244.251271623229));
#22424=CARTESIAN_POINT('Ctrl Pts',(272.242998068607,167.351822457037,244.505176818944));
#22425=CARTESIAN_POINT('Ctrl Pts',(270.925403851406,165.868758860831,244.251271623229));
#22426=CARTESIAN_POINT('Ctrl Pts',(270.12291983318,167.952002110765,244.124319025372));
#22427=CARTESIAN_POINT('Ctrl Pts',(270.853560396594,167.28114638485,244.25127162323));
#22428=CARTESIAN_POINT('Ctrl Pts',(270.194763287993,166.539614586747,244.124319025372));
#22429=CARTESIAN_POINT('Ctrl Pts',(269.46412272458,167.210470312662,243.997366427515));
#22430=CARTESIAN_POINT('Ctrl Pts',(269.46412272458,167.210470312662,243.997366427515));
#22431=CARTESIAN_POINT('Ctrl Pts',(269.46412272458,167.210470312662,243.997366427515));
#22432=CARTESIAN_POINT('Ctrl Pts',(269.284816459225,167.201349599434,244.98111745079));
#22433=CARTESIAN_POINT('Ctrl Pts',(269.284816459225,167.201349599434,244.98111745079));
#22434=CARTESIAN_POINT('Ctrl Pts',(269.284816459225,167.201349599434,244.98111745079));
#22435=CARTESIAN_POINT('Origin',(238.067118190679,151.504231246999,245.983333506556));
#22436=CARTESIAN_POINT('',(241.032274232146,152.585076330075,248.440898064434));
#22437=CARTESIAN_POINT('Origin',(241.773563242513,152.855287600844,249.055289203903));
#22438=CARTESIAN_POINT('',(237.128624750255,148.490992705803,248.440898064434));
#22439=CARTESIAN_POINT('Origin',(238.067118190679,151.504231246999,245.983333506556));
#22440=CARTESIAN_POINT('Origin',(236.894001390149,147.737683070505,249.055289203903));
#22441=CARTESIAN_POINT('Origin',(228.757252972023,138.49174626232,249.917994543901));
#22442=CARTESIAN_POINT('',(231.722409013491,139.572591345396,252.375559101779));
#22443=CARTESIAN_POINT('Origin',(232.463698023858,139.842802616165,252.989950241249));
#22444=CARTESIAN_POINT('',(227.324186103648,139.858154780476,246.442473415743));
#22445=CARTESIAN_POINT('Origin',(228.757252972023,138.49174626232,249.917994543901));
#22446=CARTESIAN_POINT('Origin',(226.965919386554,140.199756910015,245.573593133703));
#22447=CARTESIAN_POINT('Origin',(243.960011343564,155.655639048279,248.440898064434));
#22448=CARTESIAN_POINT('',(244.19463470367,156.408948683578,247.826506924964));
#22449=CARTESIAN_POINT('',(243.321882482923,155.655639048279,249.210827643822));
#22450=CARTESIAN_POINT('Origin',(243.960011343564,155.655639048279,248.440898064434));
#22451=CARTESIAN_POINT('Origin',(243.960011343564,155.655639048279,248.440898064434));
#22452=CARTESIAN_POINT('',(243.960011343564,155.655639048279,249.440898064434));
#22453=CARTESIAN_POINT('Origin',(243.960011343564,155.655639048279,248.440898064434));
#22454=CARTESIAN_POINT('Origin',(245.597924271693,159.74069839092,245.573593133703));
#22455=CARTESIAN_POINT('',(244.874185698326,160.430772645925,245.573593133703));
#22456=CARTESIAN_POINT('',(245.956190988787,159.399096261381,246.442473415743));
#22457=CARTESIAN_POINT('Origin',(245.597924271693,159.74069839092,245.573593133703));
#22458=CARTESIAN_POINT('',(246.597924271693,159.74069839092,245.573593133703));
#22459=CARTESIAN_POINT('Origin',(245.597924271693,159.74069839092,245.573593133703));
#22460=CARTESIAN_POINT('Origin',(245.597924271693,159.74069839092,245.573593133703));
#22461=CARTESIAN_POINT('Origin',(243.218722333198,155.38542777751,247.826506924964));
#22462=CARTESIAN_POINT('',(243.453345693303,156.138737412809,247.212115785495));
#22463=CARTESIAN_POINT('',(243.453345693303,156.138737412809,247.212115785495));
#22464=CARTESIAN_POINT('',(242.984098973092,154.632118142211,248.440898064434));
#22465=CARTESIAN_POINT('Origin',(243.218722333198,155.38542777751,247.826506924964));
#22466=CARTESIAN_POINT('Origin',(243.218722333198,155.38542777751,247.826506924964));
#22467=CARTESIAN_POINT('Origin',(241.773563242513,152.855287600844,249.055289203903));
#22468=CARTESIAN_POINT('',(241.501520952358,154.091695600673,247.212115785495));
#22469=CARTESIAN_POINT('Origin',(242.242809962725,154.361906871442,247.826506924964));
#22470=CARTESIAN_POINT('',(241.032274232146,152.585076330075,248.440898064434));
#22471=CARTESIAN_POINT('Origin',(242.242809962725,154.361906871442,247.826506924964));
#22472=CARTESIAN_POINT('Origin',(235.411423369415,147.197260528966,247.826506924964));
#22473=CARTESIAN_POINT('',(235.646046729521,147.950570164265,247.212115785495));
#22474=CARTESIAN_POINT('',(235.646046729521,147.950570164265,247.212115785495));
#22475=CARTESIAN_POINT('',(235.176800009309,146.443950893667,248.440898064434));
#22476=CARTESIAN_POINT('Origin',(235.411423369415,147.197260528966,247.826506924964));
#22477=CARTESIAN_POINT('Origin',(235.411423369415,147.197260528966,247.826506924964));
#22478=CARTESIAN_POINT('Origin',(232.463698023858,139.842802616165,252.989950241249));
#22479=CARTESIAN_POINT('',(233.694221988576,145.903528352129,247.212115785495));
#22480=CARTESIAN_POINT('Origin',(234.435510998943,146.173739622898,247.826506924964));
#22481=CARTESIAN_POINT('',(231.722409013491,139.572591345396,252.375559101779));
#22482=CARTESIAN_POINT('Origin',(234.435510998943,146.173739622898,247.826506924964));
#22483=CARTESIAN_POINT('Origin',(246.287998526698,160.464436964287,245.573593133703));
#22484=CARTESIAN_POINT('',(246.646265243792,160.122834834748,246.442473415743));
#22485=CARTESIAN_POINT('Ctrl Pts',(242.984098973092,154.632118142211,248.440898064434));
#22486=CARTESIAN_POINT('Ctrl Pts',(242.984098973092,154.632118142211,248.440898064434));
#22487=CARTESIAN_POINT('Ctrl Pts',(242.984098973092,154.632118142211,248.440898064434));
#22488=CARTESIAN_POINT('Ctrl Pts',(242.355256797342,155.231710055528,248.935920342198));
#22489=CARTESIAN_POINT('Ctrl Pts',(242.355256797342,155.231710055528,248.935920342198));
#22490=CARTESIAN_POINT('Ctrl Pts',(242.355256797342,155.231710055528,248.935920342198));
#22491=CARTESIAN_POINT('Ctrl Pts',(241.613967786975,154.961498784759,248.321529202729));
#22492=CARTESIAN_POINT('Ctrl Pts',(241.848591147081,155.714808420058,247.707138063259));
#22493=CARTESIAN_POINT('Ctrl Pts',(242.589880157448,155.985019690827,248.321529202729));
#22494=CARTESIAN_POINT('Ctrl Pts',(240.872678776608,154.69128751399,247.707138063259));
#22495=CARTESIAN_POINT('Ctrl Pts',(241.34192549682,156.197906784588,246.47835578432));
#22496=CARTESIAN_POINT('Ctrl Pts',(242.824503517554,156.738329326126,247.707138063259));
#22497=CARTESIAN_POINT('Ctrl Pts',(241.501520952358,154.091695600673,247.212115785495));
#22498=CARTESIAN_POINT('Ctrl Pts',(241.97076767257,155.598314871271,245.983333506556));
#22499=CARTESIAN_POINT('Ctrl Pts',(243.453345693303,156.138737412809,247.212115785495));
#22500=CARTESIAN_POINT('Ctrl Pts',(242.130363128108,153.492103687356,246.717093507731));
#22501=CARTESIAN_POINT('Ctrl Pts',(242.59960984832,154.998722957953,245.488311228792));
#22502=CARTESIAN_POINT('Ctrl Pts',(244.082187869053,155.539145499492,246.717093507731));
#22503=CARTESIAN_POINT('Ctrl Pts',(242.871652138475,153.762314958125,247.3314846472));
#22504=CARTESIAN_POINT('Ctrl Pts',(243.106275498581,154.515624593424,246.717093507731));
#22505=CARTESIAN_POINT('Ctrl Pts',(243.847564508947,154.785835864193,247.3314846472));
#22506=CARTESIAN_POINT('Ctrl Pts',(243.612941148842,154.032526228894,247.94587578667));
#22507=CARTESIAN_POINT('Ctrl Pts',(243.612941148842,154.032526228894,247.94587578667));
#22508=CARTESIAN_POINT('Ctrl Pts',(243.612941148842,154.032526228894,247.94587578667));
#22509=CARTESIAN_POINT('Ctrl Pts',(242.984098973092,154.632118142211,248.440898064434));
#22510=CARTESIAN_POINT('Ctrl Pts',(242.984098973092,154.632118142211,248.440898064434));
#22511=CARTESIAN_POINT('Ctrl Pts',(242.984098973092,154.632118142211,248.440898064434));
#22512=CARTESIAN_POINT('Ctrl Pts',(235.176800009309,146.443950893667,248.440898064434));
#22513=CARTESIAN_POINT('Ctrl Pts',(235.176800009309,146.443950893667,248.440898064434));
#22514=CARTESIAN_POINT('Ctrl Pts',(235.176800009309,146.443950893667,248.440898064434));
#22515=CARTESIAN_POINT('Ctrl Pts',(234.547957833559,147.043542806985,248.935920342198));
#22516=CARTESIAN_POINT('Ctrl Pts',(234.547957833559,147.043542806985,248.935920342198));
#22517=CARTESIAN_POINT('Ctrl Pts',(234.547957833559,147.043542806985,248.935920342198));
#22518=CARTESIAN_POINT('Ctrl Pts',(233.806668823193,146.773331536215,248.321529202729));
#22519=CARTESIAN_POINT('Ctrl Pts',(234.041292183298,147.526641171514,247.707138063259));
#22520=CARTESIAN_POINT('Ctrl Pts',(234.782581193665,147.796852442283,248.321529202729));
#22521=CARTESIAN_POINT('Ctrl Pts',(233.065379812826,146.503120265446,247.707138063259));
#22522=CARTESIAN_POINT('Ctrl Pts',(233.534626533037,148.009739536044,246.47835578432));
#22523=CARTESIAN_POINT('Ctrl Pts',(235.017204553771,148.550162077582,247.707138063259));
#22524=CARTESIAN_POINT('Ctrl Pts',(233.694221988576,145.903528352129,247.212115785495));
#22525=CARTESIAN_POINT('Ctrl Pts',(234.163468708787,147.410147622727,245.983333506556));
#22526=CARTESIAN_POINT('Ctrl Pts',(235.646046729521,147.950570164265,247.212115785495));
#22527=CARTESIAN_POINT('Ctrl Pts',(234.323064164326,145.303936438812,246.717093507731));
#22528=CARTESIAN_POINT('Ctrl Pts',(234.792310884537,146.81055570941,245.488311228792));
#22529=CARTESIAN_POINT('Ctrl Pts',(236.274888905271,147.350978250948,246.717093507731));
#22530=CARTESIAN_POINT('Ctrl Pts',(235.064353174692,145.574147709581,247.3314846472));
#22531=CARTESIAN_POINT('Ctrl Pts',(235.298976534798,146.32745734488,246.717093507731));
#22532=CARTESIAN_POINT('Ctrl Pts',(236.040265545165,146.597668615649,247.3314846472));
#22533=CARTESIAN_POINT('Ctrl Pts',(235.805642185059,145.84435898035,247.94587578667));
#22534=CARTESIAN_POINT('Ctrl Pts',(235.805642185059,145.84435898035,247.94587578667));
#22535=CARTESIAN_POINT('Ctrl Pts',(235.805642185059,145.84435898035,247.94587578667));
#22536=CARTESIAN_POINT('Ctrl Pts',(235.176800009309,146.443950893667,248.440898064434));
#22537=CARTESIAN_POINT('Ctrl Pts',(235.176800009309,146.443950893667,248.440898064434));
#22538=CARTESIAN_POINT('Ctrl Pts',(235.176800009309,146.443950893667,248.440898064434));
#27767=UNCERTAINTY_MEASURE_WITH_UNIT(LENGTH_MEASURE(0.01),#27808,
'DISTANCE_ACCURACY_VALUE',
'Maximum model space distance between geometric entities at asserted c
onnectivities');
#27778=UNCERTAINTY_MEASURE_WITH_UNIT(LENGTH_MEASURE(0.01),#27808,
'DISTANCE_ACCURACY_VALUE',
'Maximum model space distance between geometric entities at asserted c
onnectivities');
#27796=(
GEOMETRIC_REPRESENTATION_CONTEXT(3)
GLOBAL_UNCERTAINTY_ASSIGNED_CONTEXT((#27767))
GLOBAL_UNIT_ASSIGNED_CONTEXT((#27808,#27810,#27811))
REPRESENTATION_CONTEXT('','3D')
);
#27807=(
GEOMETRIC_REPRESENTATION_CONTEXT(3)
GLOBAL_UNCERTAINTY_ASSIGNED_CONTEXT((#27778))
GLOBAL_UNIT_ASSIGNED_CONTEXT((#27808,#27810,#27811))
REPRESENTATION_CONTEXT('','3D')
);
#27808=(
LENGTH_UNIT()
NAMED_UNIT(*)
SI_UNIT(.MILLI.,.METRE.)
);
#27810=(
NAMED_UNIT(*)
PLANE_ANGLE_UNIT()
SI_UNIT($,.RADIAN.)
);
#27811=(
NAMED_UNIT(*)
SI_UNIT($,.STERADIAN.)
SOLID_ANGLE_UNIT()
);
#27829=SHAPE_DEFINITION_REPRESENTATION(#27862,#27916);
#27862=PRODUCT_DEFINITION_SHAPE('',$,#27945);
#27916=SHAPE_REPRESENTATION('',(#13302),#27796);
#27927=PRODUCT_DEFINITION_CONTEXT('part definition',#28013,'design');
#27945=PRODUCT_DEFINITION('Retaining Clips','Retaining Clips',#27973,#27927);
#27973=PRODUCT_DEFINITION_FORMATION('',$,#28032);
#28013=APPLICATION_CONTEXT('Managed model based 3d engineering');
#28014=PRODUCT_CONTEXT('part definition',#28013,'mechanical');
#28032=PRODUCT('Retaining Clips','Retaining Clips',$,(#28014));
#28064=COLOUR_RGB('Sky Blue',0.24,0.69,0.87);
#28065=FILL_AREA_STYLE_COLOUR('',#28064);
#28066=FILL_AREA_STYLE('',(#28065));
#28067=SURFACE_STYLE_FILL_AREA(#28066);
#28068=SURFACE_SIDE_STYLE('',(#28067));
#28069=SURFACE_STYLE_USAGE(.BOTH.,#28068);
#28070=PRESENTATION_STYLE_ASSIGNMENT((#28069));
ENDSEC;
END-ISO-10303-21;
